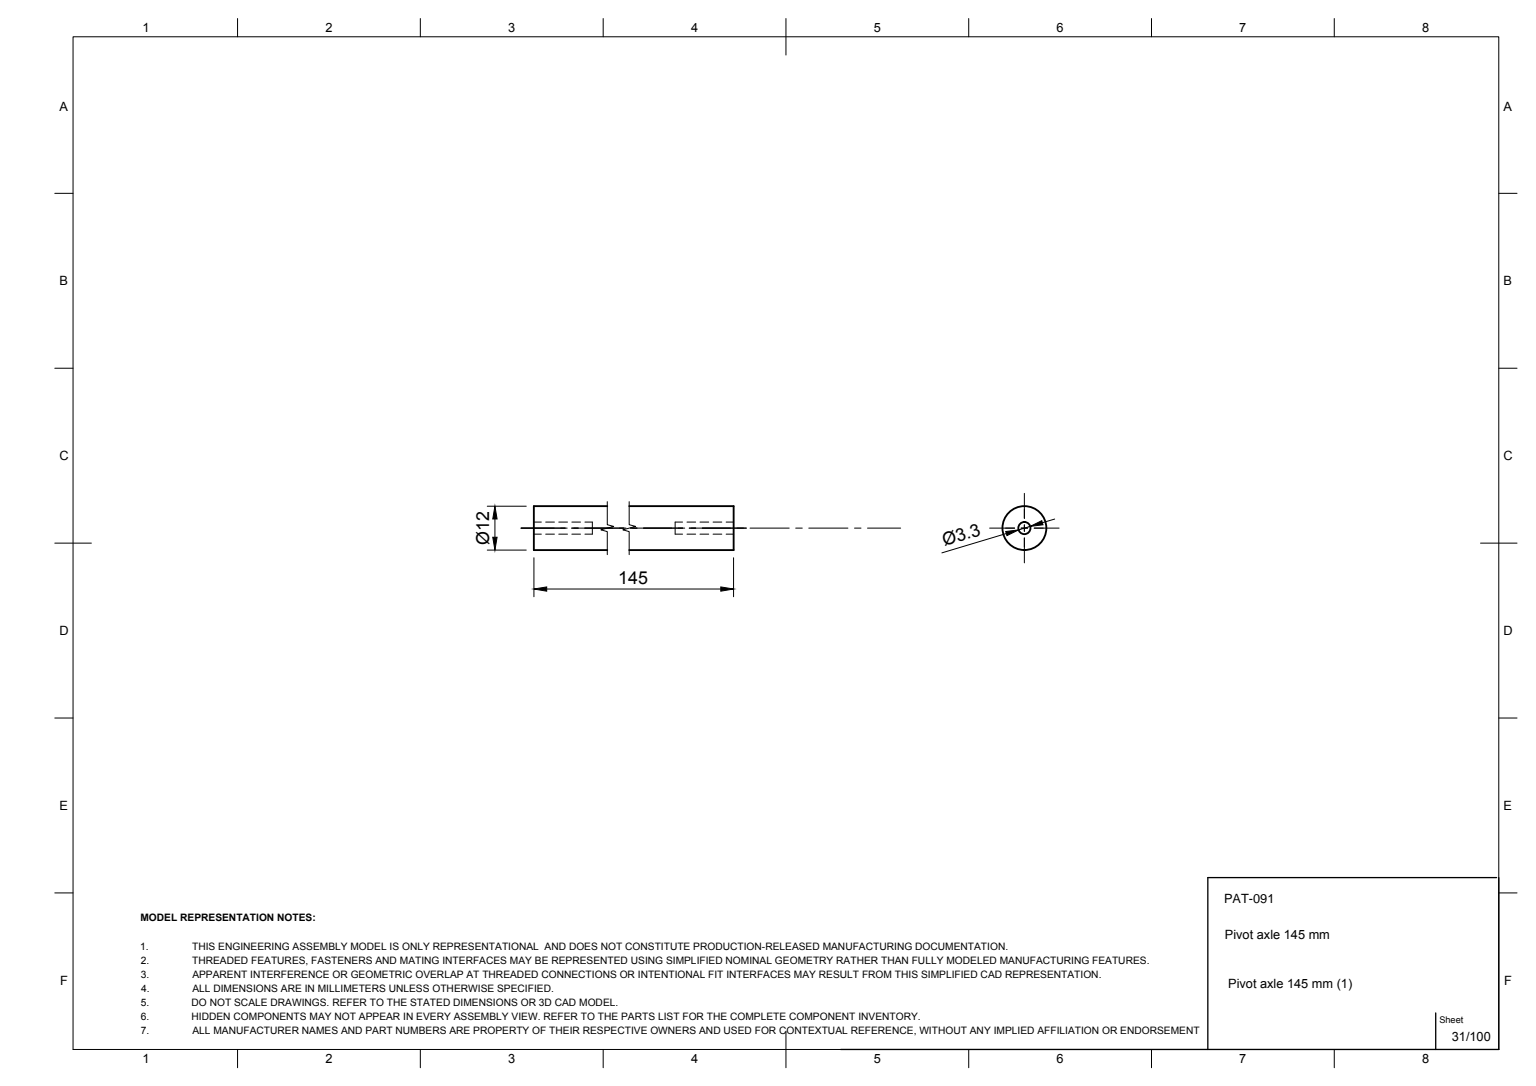
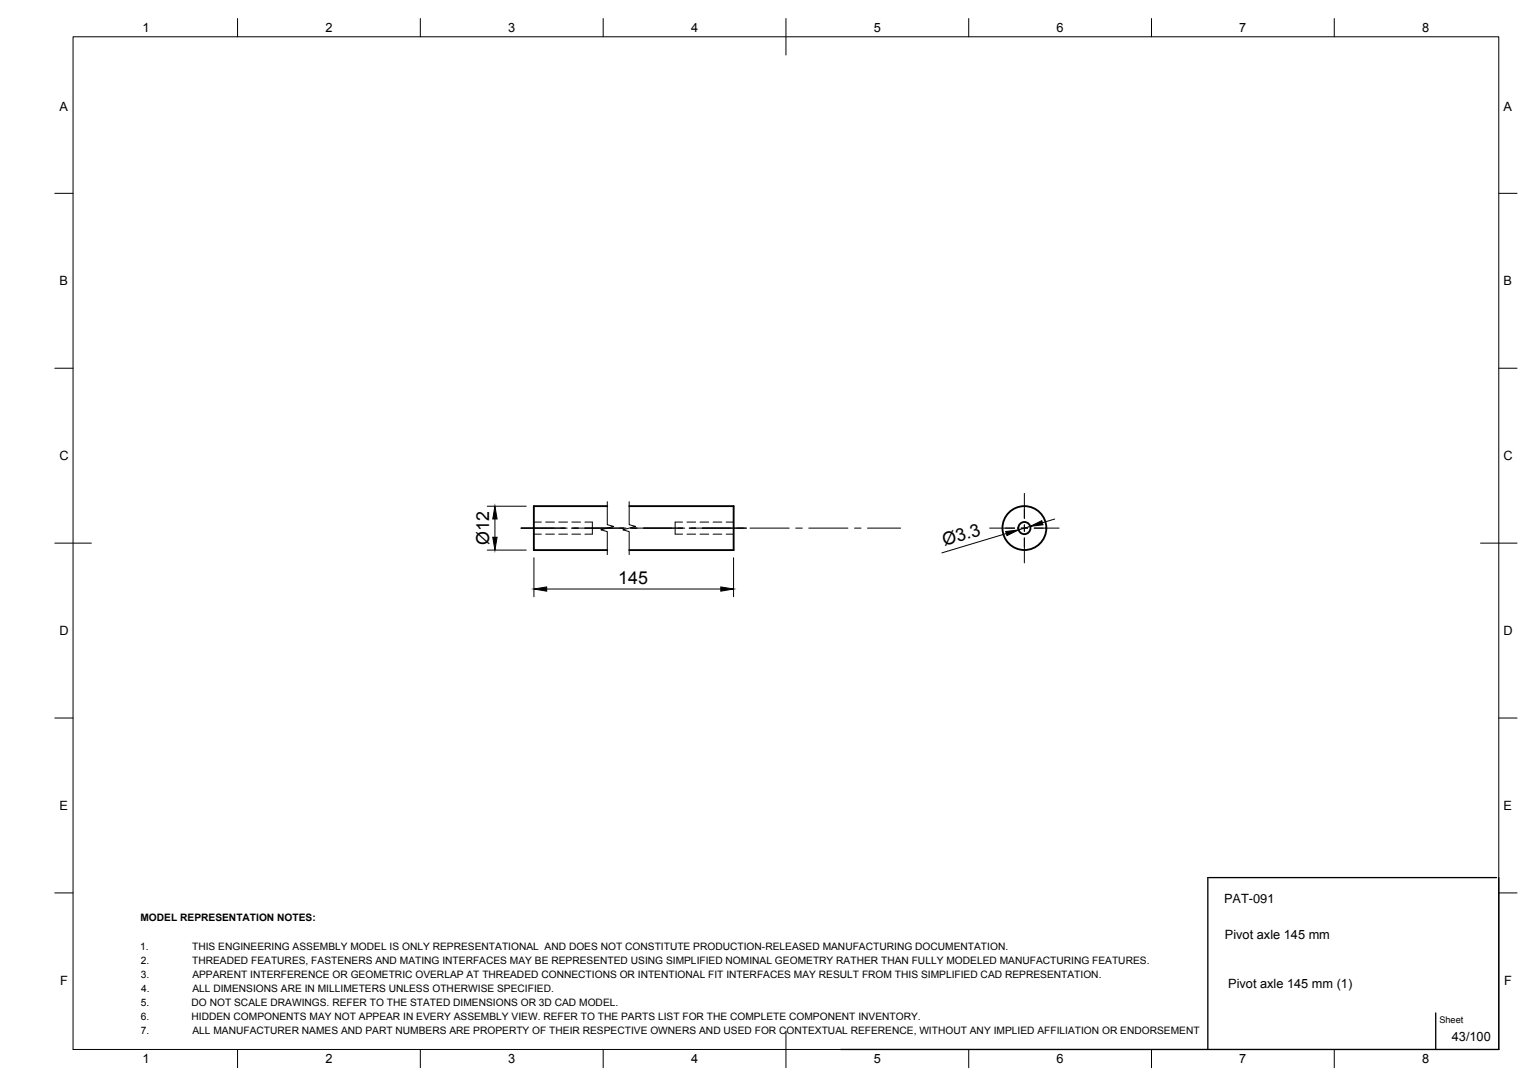
ISO-10303-21;
HEADER;
/* Generated by software containing ST-Developer
 * from STEP Tools, Inc. (www.steptools.com) 
 */

FILE_DESCRIPTION(
/* description */ ('PAT-091'),
/* implementation_level */ '2;1');

FILE_NAME(
/* name */ 'Pivot axle 145 mm (1).step',
/* time_stamp */ '2026-10-27T15:34:44-07:00',
/* author */ (''),
/* organization */ (''),
/* preprocessor_version */ 'ST-DEVELOPER v20.2',
/* originating_system */ 'Autodesk Translation Framework v15.17.0.0',
/* authorisation */ '');

FILE_SCHEMA (('AUTOMOTIVE_DESIGN { 1 0 10303 214 3 1 1 }'));
ENDSEC;

DATA;
#10=MECHANICAL_DESIGN_GEOMETRIC_PRESENTATION_REPRESENTATION('',(#1006),#25100);
#786=SHAPE_REPRESENTATION_RELATIONSHIP('SRR','None',#25549,#896);
#896=ADVANCED_BREP_SHAPE_REPRESENTATION('',(#1128),#25019);
#1006=STYLED_ITEM('',(#26191),#1128);
#1128=MANIFOLD_SOLID_BREP('Body1',#13285);
#1418=FACE_BOUND('',#3395,.T.);
#1419=FACE_BOUND('',#3397,.T.);
#1807=PLANE('',#15204);
#1808=PLANE('',#15208);
#1809=PLANE('',#15212);
#1810=PLANE('',#15213);
#2368=FACE_OUTER_BOUND('',#3389,.T.);
#2369=FACE_OUTER_BOUND('',#3390,.T.);
#2370=FACE_OUTER_BOUND('',#3391,.T.);
#2371=FACE_OUTER_BOUND('',#3392,.T.);
#2372=FACE_OUTER_BOUND('',#3393,.T.);
#2373=FACE_OUTER_BOUND('',#3394,.T.);
#2374=FACE_OUTER_BOUND('',#3396,.T.);
#3389=EDGE_LOOP('',(#10254,#10255,#10256,#10257));
#3390=EDGE_LOOP('',(#10258));
#3391=EDGE_LOOP('',(#10259,#10260,#10261,#10262));
#3392=EDGE_LOOP('',(#10263));
#3393=EDGE_LOOP('',(#10264,#10265,#10266,#10267));
#3394=EDGE_LOOP('',(#10268));
#3395=EDGE_LOOP('',(#10269));
#3396=EDGE_LOOP('',(#10270));
#3397=EDGE_LOOP('',(#10271));
#4492=LINE('',#22415,#5232);
#4493=LINE('',#22422,#5233);
#4494=LINE('',#22429,#5234);
#5232=VECTOR('',#18072,0.164999999999999);
#5233=VECTOR('',#18081,0.164999999999999);
#5234=VECTOR('',#18090,0.600000000000001);
#5875=CIRCLE('',#15202,0.164999999999999);
#5876=CIRCLE('',#15203,0.164999999999999);
#5877=CIRCLE('',#15206,0.164999999999999);
#5878=CIRCLE('',#15207,0.164999999999999);
#5879=CIRCLE('',#15210,0.600000000000001);
#5880=CIRCLE('',#15211,0.600000000000001);
#6808=VERTEX_POINT('',#22412);
#6809=VERTEX_POINT('',#22414);
#6810=VERTEX_POINT('',#22419);
#6811=VERTEX_POINT('',#22421);
#6812=VERTEX_POINT('',#22426);
#6813=VERTEX_POINT('',#22428);
#8062=EDGE_CURVE('',#6808,#6808,#5875,.T.);
#8063=EDGE_CURVE('',#6808,#6809,#4492,.T.);
#8064=EDGE_CURVE('',#6809,#6809,#5876,.T.);
#8065=EDGE_CURVE('',#6810,#6810,#5877,.T.);
#8066=EDGE_CURVE('',#6810,#6811,#4493,.T.);
#8067=EDGE_CURVE('',#6811,#6811,#5878,.T.);
#8068=EDGE_CURVE('',#6812,#6812,#5879,.T.);
#8069=EDGE_CURVE('',#6812,#6813,#4494,.T.);
#8070=EDGE_CURVE('',#6813,#6813,#5880,.T.);
#10254=ORIENTED_EDGE('',*,*,#8062,.F.);
#10255=ORIENTED_EDGE('',*,*,#8063,.T.);
#10256=ORIENTED_EDGE('',*,*,#8064,.F.);
#10257=ORIENTED_EDGE('',*,*,#8063,.F.);
#10258=ORIENTED_EDGE('',*,*,#8062,.T.);
#10259=ORIENTED_EDGE('',*,*,#8065,.F.);
#10260=ORIENTED_EDGE('',*,*,#8066,.T.);
#10261=ORIENTED_EDGE('',*,*,#8067,.T.);
#10262=ORIENTED_EDGE('',*,*,#8066,.F.);
#10263=ORIENTED_EDGE('',*,*,#8067,.F.);
#10264=ORIENTED_EDGE('',*,*,#8068,.F.);
#10265=ORIENTED_EDGE('',*,*,#8069,.T.);
#10266=ORIENTED_EDGE('',*,*,#8070,.T.);
#10267=ORIENTED_EDGE('',*,*,#8069,.F.);
#10268=ORIENTED_EDGE('',*,*,#8068,.T.);
#10269=ORIENTED_EDGE('',*,*,#8064,.T.);
#10270=ORIENTED_EDGE('',*,*,#8070,.F.);
#10271=ORIENTED_EDGE('',*,*,#8065,.T.);
#12205=CYLINDRICAL_SURFACE('',#15201,0.164999999999999);
#12206=CYLINDRICAL_SURFACE('',#15205,0.164999999999999);
#12207=CYLINDRICAL_SURFACE('',#15209,0.600000000000001);
#12735=ADVANCED_FACE('',(#2368),#12205,.F.);
#12736=ADVANCED_FACE('',(#2369),#1807,.T.);
#12737=ADVANCED_FACE('',(#2370),#12206,.F.);
#12738=ADVANCED_FACE('',(#2371),#1808,.F.);
#12739=ADVANCED_FACE('',(#2372),#12207,.T.);
#12740=ADVANCED_FACE('',(#2373,#1418),#1809,.T.);
#12741=ADVANCED_FACE('',(#2374,#1419),#1810,.F.);
#13285=CLOSED_SHELL('',(#12735,#12736,#12737,#12738,#12739,#12740,#12741));
#15200=AXIS2_PLACEMENT_3D('',#22410,#18066,#18067);
#15201=AXIS2_PLACEMENT_3D('',#22411,#18068,#18069);
#15202=AXIS2_PLACEMENT_3D('',#22413,#18070,#18071);
#15203=AXIS2_PLACEMENT_3D('',#22416,#18073,#18074);
#15204=AXIS2_PLACEMENT_3D('',#22417,#18075,#18076);
#15205=AXIS2_PLACEMENT_3D('',#22418,#18077,#18078);
#15206=AXIS2_PLACEMENT_3D('',#22420,#18079,#18080);
#15207=AXIS2_PLACEMENT_3D('',#22423,#18082,#18083);
#15208=AXIS2_PLACEMENT_3D('',#22424,#18084,#18085);
#15209=AXIS2_PLACEMENT_3D('',#22425,#18086,#18087);
#15210=AXIS2_PLACEMENT_3D('',#22427,#18088,#18089);
#15211=AXIS2_PLACEMENT_3D('',#22430,#18091,#18092);
#15212=AXIS2_PLACEMENT_3D('',#22431,#18093,#18094);
#15213=AXIS2_PLACEMENT_3D('',#22432,#18095,#18096);
#18066=DIRECTION('axis',(0.,0.,1.));
#18067=DIRECTION('refdir',(1.,0.,0.));
#18068=DIRECTION('center_axis',(0.,1.,0.));
#18069=DIRECTION('ref_axis',(1.,0.,0.));
#18070=DIRECTION('center_axis',(0.,1.,0.));
#18071=DIRECTION('ref_axis',(1.,0.,0.));
#18072=DIRECTION('',(0.,1.,0.));
#18073=DIRECTION('center_axis',(0.,-1.,0.));
#18074=DIRECTION('ref_axis',(1.,0.,0.));
#18075=DIRECTION('center_axis',(0.,1.,0.));
#18076=DIRECTION('ref_axis',(1.,0.,0.));
#18077=DIRECTION('center_axis',(0.,1.,0.));
#18078=DIRECTION('ref_axis',(1.,0.,0.));
#18079=DIRECTION('center_axis',(0.,1.,0.));
#18080=DIRECTION('ref_axis',(1.,0.,0.));
#18081=DIRECTION('',(0.,1.,0.));
#18082=DIRECTION('center_axis',(0.,1.,0.));
#18083=DIRECTION('ref_axis',(1.,0.,0.));
#18084=DIRECTION('center_axis',(0.,1.,0.));
#18085=DIRECTION('ref_axis',(1.,0.,0.));
#18086=DIRECTION('center_axis',(0.,1.,0.));
#18087=DIRECTION('ref_axis',(1.,0.,0.));
#18088=DIRECTION('center_axis',(0.,1.,0.));
#18089=DIRECTION('ref_axis',(1.,0.,0.));
#18090=DIRECTION('',(0.,-1.,0.));
#18091=DIRECTION('center_axis',(0.,1.,0.));
#18092=DIRECTION('ref_axis',(1.,0.,0.));
#18093=DIRECTION('center_axis',(0.,1.,0.));
#18094=DIRECTION('ref_axis',(1.,0.,0.));
#18095=DIRECTION('center_axis',(0.,1.,0.));
#18096=DIRECTION('ref_axis',(1.,0.,0.));
#22410=CARTESIAN_POINT('',(0.,0.,0.));
#22411=CARTESIAN_POINT('Origin',(38.7298334620742,6.9,3.));
#22412=CARTESIAN_POINT('',(38.5648334620742,6.9,3.));
#22413=CARTESIAN_POINT('Origin',(38.7298334620742,6.9,3.));
#22414=CARTESIAN_POINT('',(38.5648334620742,8.5,3.));
#22415=CARTESIAN_POINT('',(38.5648334620742,6.9,3.));
#22416=CARTESIAN_POINT('Origin',(38.7298334620742,8.5,3.));
#22417=CARTESIAN_POINT('Origin',(38.7298334620742,6.9,3.));
#22418=CARTESIAN_POINT('Origin',(38.7298334620742,-6.1,3.));
#22419=CARTESIAN_POINT('',(38.5648334620742,-6.,3.));
#22420=CARTESIAN_POINT('Origin',(38.7298334620742,-6.,3.));
#22421=CARTESIAN_POINT('',(38.5648334620742,-4.4,3.));
#22422=CARTESIAN_POINT('',(38.5648334620742,-6.1,3.));
#22423=CARTESIAN_POINT('Origin',(38.7298334620742,-4.4,3.));
#22424=CARTESIAN_POINT('Origin',(38.7298334620742,-4.4,3.));
#22425=CARTESIAN_POINT('Origin',(38.7298334620742,-6.,3.));
#22426=CARTESIAN_POINT('',(38.1298334620742,8.5,3.));
#22427=CARTESIAN_POINT('Origin',(38.7298334620742,8.5,3.));
#22428=CARTESIAN_POINT('',(38.1298334620742,-6.,3.));
#22429=CARTESIAN_POINT('',(38.1298334620742,-6.,3.));
#22430=CARTESIAN_POINT('Origin',(38.7298334620742,-6.,3.));
#22431=CARTESIAN_POINT('Origin',(38.7298334620742,8.5,3.));
#22432=CARTESIAN_POINT('Origin',(38.7298334620742,-6.,3.));
#24898=UNCERTAINTY_MEASURE_WITH_UNIT(LENGTH_MEASURE(0.001),#25101,
'DISTANCE_ACCURACY_VALUE',
'Maximum model space distance between geometric entities at asserted c
onnectivities');
#24979=UNCERTAINTY_MEASURE_WITH_UNIT(LENGTH_MEASURE(0.001),#25101,
'DISTANCE_ACCURACY_VALUE',
'Maximum model space distance between geometric entities at asserted c
onnectivities');
#25019=(
GEOMETRIC_REPRESENTATION_CONTEXT(3)
GLOBAL_UNCERTAINTY_ASSIGNED_CONTEXT((#24898))
GLOBAL_UNIT_ASSIGNED_CONTEXT((#25101,#25103,#25104))
REPRESENTATION_CONTEXT('','3D')
);
#25100=(
GEOMETRIC_REPRESENTATION_CONTEXT(3)
GLOBAL_UNCERTAINTY_ASSIGNED_CONTEXT((#24979))
GLOBAL_UNIT_ASSIGNED_CONTEXT((#25101,#25103,#25104))
REPRESENTATION_CONTEXT('','3D')
);
#25101=(
LENGTH_UNIT()
NAMED_UNIT(*)
SI_UNIT(.CENTI.,.METRE.)
);
#25103=(
NAMED_UNIT(*)
PLANE_ANGLE_UNIT()
SI_UNIT($,.RADIAN.)
);
#25104=(
NAMED_UNIT(*)
SI_UNIT($,.STERADIAN.)
SOLID_ANGLE_UNIT()
);
#25144=SHAPE_DEFINITION_REPRESENTATION(#25264,#25549);
#25264=PRODUCT_DEFINITION_SHAPE('',$,#25670);
#25549=SHAPE_REPRESENTATION('',(#15200),#25019);
#25630=PRODUCT_DEFINITION_CONTEXT('part definition',#25992,'design');
#25670=PRODUCT_DEFINITION('Pivot axle 145 mm (1)','Pivot axle 145 mm (1)',
#25790,#25630);
#25790=PRODUCT_DEFINITION_FORMATION('',$,#26033);
#25992=APPLICATION_CONTEXT(
'Core Data for Automotive Mechanical Design Process');
#25993=PRODUCT_CONTEXT('part definition',#25992,'mechanical');
#26033=PRODUCT('Pivot axle 145 mm (1)','Pivot axle 145 mm (1)',
'Pivot axle 145 mm (1)',(#25993));
#26185=COLOUR_RGB('Grey',0.48,0.52,0.57);
#26186=FILL_AREA_STYLE_COLOUR('',#26185);
#26187=FILL_AREA_STYLE('',(#26186));
#26188=SURFACE_STYLE_FILL_AREA(#26187);
#26189=SURFACE_SIDE_STYLE('',(#26188));
#26190=SURFACE_STYLE_USAGE(.BOTH.,#26189);
#26191=PRESENTATION_STYLE_ASSIGNMENT((#26190));
ENDSEC;
END-ISO-10303-21;
